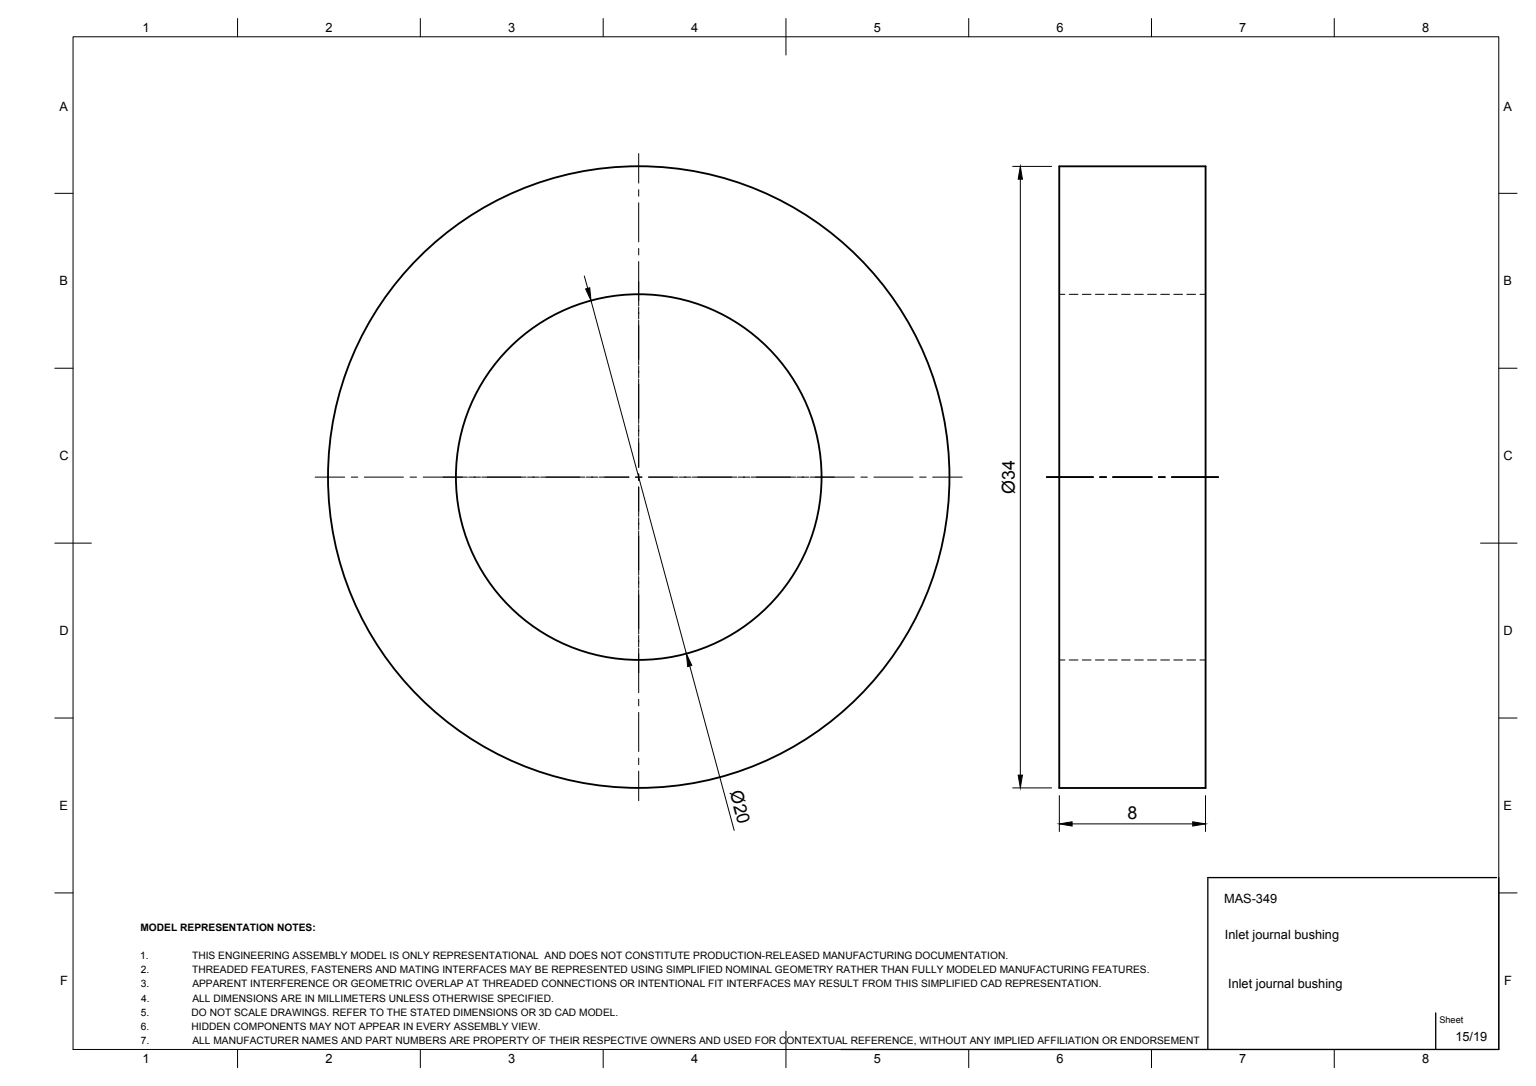
ISO-10303-21;
HEADER;
/* Generated by software containing ST-Developer
 * from STEP Tools, Inc. (www.steptools.com) 
 */

FILE_DESCRIPTION(
/* description */ ('Independent two-stage semi-open centrifugal-pump CAD. Shared impeller
s, open-machinable return casings, removable diaphragms, bronze wear/j
ournal rings, volume-preserving seal instances, retained keyed shaft, 
opposed mechanical face rings and partly threaded tie hardware. Native
 shaft rotation. Geometric topology/clearance only; flow/head/efficien
cy, pressure, cavitation, balance, preload, face loading and secondary
 seal fits/bonds, material/thermal/tolerance selection and life unassi
gned. External drive, coupling, anchors and piping bolts omitted.'),
/* implementation_level */ '2;1');

FILE_NAME(
/* name */ 'Inlet journal bushing.step',
/* time_stamp */ '2026-11-08T18:06:32-08:00',
/* author */ (''),
/* organization */ (''),
/* preprocessor_version */ 'ST-DEVELOPER v20.2',
/* originating_system */ 'Autodesk Translation Framework v15.17.0.0',
/* authorisation */ '');

FILE_SCHEMA (('AUTOMOTIVE_DESIGN { 1 0 10303 214 3 1 1 }'));
ENDSEC;

DATA;
#10=MECHANICAL_DESIGN_GEOMETRIC_PRESENTATION_REPRESENTATION('',(#404),#16687);
#366=SHAPE_REPRESENTATION_RELATIONSHIP('SRR','None',#16775,#385);
#385=ADVANCED_BREP_SHAPE_REPRESENTATION('',(#423),#16679);
#404=STYLED_ITEM('',(#16875),#423);
#423=MANIFOLD_SOLID_BREP('Body1',#6123);
#541=FACE_BOUND('',#1430,.T.);
#542=FACE_BOUND('',#1432,.T.);
#657=PLANE('',#6858);
#658=PLANE('',#6859);
#970=FACE_OUTER_BOUND('',#1427,.T.);
#971=FACE_OUTER_BOUND('',#1428,.T.);
#972=FACE_OUTER_BOUND('',#1429,.T.);
#973=FACE_OUTER_BOUND('',#1431,.T.);
#1427=EDGE_LOOP('',(#5293,#5294,#5295,#5296));
#1428=EDGE_LOOP('',(#5297,#5298,#5299,#5300));
#1429=EDGE_LOOP('',(#5301));
#1430=EDGE_LOOP('',(#5302));
#1431=EDGE_LOOP('',(#5303));
#1432=EDGE_LOOP('',(#5304));
#1810=LINE('',#15150,#2179);
#1811=LINE('',#15156,#2180);
#2179=VECTOR('',#8322,1.);
#2180=VECTOR('',#8329,1.7);
#2462=CIRCLE('',#6853,1.);
#2463=CIRCLE('',#6854,1.);
#2464=CIRCLE('',#6856,1.7);
#2465=CIRCLE('',#6857,1.7);
#2965=VERTEX_POINT('',#15147);
#2966=VERTEX_POINT('',#15149);
#2967=VERTEX_POINT('',#15153);
#2968=VERTEX_POINT('',#15155);
#3756=EDGE_CURVE('',#2965,#2965,#2462,.T.);
#3757=EDGE_CURVE('',#2965,#2966,#1810,.T.);
#3758=EDGE_CURVE('',#2966,#2966,#2463,.T.);
#3759=EDGE_CURVE('',#2967,#2967,#2464,.T.);
#3760=EDGE_CURVE('',#2967,#2968,#1811,.T.);
#3761=EDGE_CURVE('',#2968,#2968,#2465,.T.);
#5293=ORIENTED_EDGE('',*,*,#3756,.F.);
#5294=ORIENTED_EDGE('',*,*,#3757,.T.);
#5295=ORIENTED_EDGE('',*,*,#3758,.T.);
#5296=ORIENTED_EDGE('',*,*,#3757,.F.);
#5297=ORIENTED_EDGE('',*,*,#3759,.F.);
#5298=ORIENTED_EDGE('',*,*,#3760,.T.);
#5299=ORIENTED_EDGE('',*,*,#3761,.T.);
#5300=ORIENTED_EDGE('',*,*,#3760,.F.);
#5301=ORIENTED_EDGE('',*,*,#3759,.T.);
#5302=ORIENTED_EDGE('',*,*,#3756,.T.);
#5303=ORIENTED_EDGE('',*,*,#3761,.F.);
#5304=ORIENTED_EDGE('',*,*,#3758,.F.);
#5734=CYLINDRICAL_SURFACE('',#6852,1.);
#5735=CYLINDRICAL_SURFACE('',#6855,1.7);
#6049=ADVANCED_FACE('',(#970),#5734,.F.);
#6050=ADVANCED_FACE('',(#971),#5735,.T.);
#6051=ADVANCED_FACE('',(#972,#541),#657,.T.);
#6052=ADVANCED_FACE('',(#973,#542),#658,.F.);
#6123=CLOSED_SHELL('',(#6049,#6050,#6051,#6052));
#6851=AXIS2_PLACEMENT_3D('',#15145,#8316,#8317);
#6852=AXIS2_PLACEMENT_3D('',#15146,#8318,#8319);
#6853=AXIS2_PLACEMENT_3D('',#15148,#8320,#8321);
#6854=AXIS2_PLACEMENT_3D('',#15151,#8323,#8324);
#6855=AXIS2_PLACEMENT_3D('',#15152,#8325,#8326);
#6856=AXIS2_PLACEMENT_3D('',#15154,#8327,#8328);
#6857=AXIS2_PLACEMENT_3D('',#15157,#8330,#8331);
#6858=AXIS2_PLACEMENT_3D('',#15158,#8332,#8333);
#6859=AXIS2_PLACEMENT_3D('',#15159,#8334,#8335);
#8316=DIRECTION('axis',(0.,0.,1.));
#8317=DIRECTION('refdir',(1.,0.,0.));
#8318=DIRECTION('center_axis',(0.,0.,1.));
#8319=DIRECTION('ref_axis',(1.,0.,0.));
#8320=DIRECTION('center_axis',(0.,0.,-1.));
#8321=DIRECTION('ref_axis',(1.,0.,0.));
#8322=DIRECTION('',(0.,0.,-1.));
#8323=DIRECTION('center_axis',(0.,0.,-1.));
#8324=DIRECTION('ref_axis',(1.,0.,0.));
#8325=DIRECTION('center_axis',(0.,0.,1.));
#8326=DIRECTION('ref_axis',(1.,0.,0.));
#8327=DIRECTION('center_axis',(0.,0.,1.));
#8328=DIRECTION('ref_axis',(1.,0.,0.));
#8329=DIRECTION('',(0.,0.,-1.));
#8330=DIRECTION('center_axis',(0.,0.,1.));
#8331=DIRECTION('ref_axis',(1.,0.,0.));
#8332=DIRECTION('center_axis',(0.,0.,1.));
#8333=DIRECTION('ref_axis',(1.,0.,0.));
#8334=DIRECTION('center_axis',(0.,0.,1.));
#8335=DIRECTION('ref_axis',(1.,0.,0.));
#15145=CARTESIAN_POINT('',(0.,0.,0.));
#15146=CARTESIAN_POINT('Origin',(0.,0.,0.));
#15147=CARTESIAN_POINT('',(-1.,-1.22464679914735E-16,0.8));
#15148=CARTESIAN_POINT('Origin',(0.,0.,0.8));
#15149=CARTESIAN_POINT('',(-1.,-1.22464679914735E-16,0.));
#15150=CARTESIAN_POINT('',(-1.,-1.22464679914735E-16,0.));
#15151=CARTESIAN_POINT('Origin',(0.,0.,0.));
#15152=CARTESIAN_POINT('Origin',(0.,0.,0.));
#15153=CARTESIAN_POINT('',(-1.7,-2.0818995585505E-16,0.8));
#15154=CARTESIAN_POINT('Origin',(0.,0.,0.8));
#15155=CARTESIAN_POINT('',(-1.7,-2.0818995585505E-16,0.));
#15156=CARTESIAN_POINT('',(-1.7,-2.0818995585505E-16,0.));
#15157=CARTESIAN_POINT('Origin',(0.,0.,0.));
#15158=CARTESIAN_POINT('Origin',(0.,0.,0.8));
#15159=CARTESIAN_POINT('Origin',(0.,0.,0.));
#16658=UNCERTAINTY_MEASURE_WITH_UNIT(LENGTH_MEASURE(0.001),#16688,
'DISTANCE_ACCURACY_VALUE',
'Maximum model space distance between geometric entities at asserted c
onnectivities');
#16666=UNCERTAINTY_MEASURE_WITH_UNIT(LENGTH_MEASURE(0.001),#16688,
'DISTANCE_ACCURACY_VALUE',
'Maximum model space distance between geometric entities at asserted c
onnectivities');
#16679=(
GEOMETRIC_REPRESENTATION_CONTEXT(3)
GLOBAL_UNCERTAINTY_ASSIGNED_CONTEXT((#16658))
GLOBAL_UNIT_ASSIGNED_CONTEXT((#16688,#16690,#16691))
REPRESENTATION_CONTEXT('','3D')
);
#16687=(
GEOMETRIC_REPRESENTATION_CONTEXT(3)
GLOBAL_UNCERTAINTY_ASSIGNED_CONTEXT((#16666))
GLOBAL_UNIT_ASSIGNED_CONTEXT((#16688,#16690,#16691))
REPRESENTATION_CONTEXT('','3D')
);
#16688=(
LENGTH_UNIT()
NAMED_UNIT(*)
SI_UNIT(.CENTI.,.METRE.)
);
#16690=(
NAMED_UNIT(*)
PLANE_ANGLE_UNIT()
SI_UNIT($,.RADIAN.)
);
#16691=(
NAMED_UNIT(*)
SI_UNIT($,.STERADIAN.)
SOLID_ANGLE_UNIT()
);
#16704=SHAPE_DEFINITION_REPRESENTATION(#16724,#16775);
#16724=PRODUCT_DEFINITION_SHAPE('',$,#16796);
#16775=SHAPE_REPRESENTATION('',(#6851),#16679);
#16783=PRODUCT_DEFINITION_CONTEXT('part definition',#16845,'design');
#16796=PRODUCT_DEFINITION('Inlet journal bushing',
'Inlet journal bushing',#16816,#16783);
#16816=PRODUCT_DEFINITION_FORMATION('',$,#16859);
#16845=APPLICATION_CONTEXT(
'Core Data for Automotive Mechanical Design Process');
#16846=PRODUCT_CONTEXT('part definition',#16845,'mechanical');
#16859=PRODUCT('Inlet journal bushing','Inlet journal bushing',$,(#16846));
#16875=PRESENTATION_STYLE_ASSIGNMENT((#16890));
#16890=SURFACE_STYLE_USAGE(.BOTH.,#16905);
#16905=SURFACE_SIDE_STYLE('',(#16920));
#16920=SURFACE_STYLE_FILL_AREA(#16935);
#16935=FILL_AREA_STYLE('Journal gray',(#16950));
#16950=FILL_AREA_STYLE_COLOUR('Journal gray',#16965);
#16965=COLOUR_RGB('Journal gray',0.725490196078431,0.752941176470588,0.792156862745098);
ENDSEC;
END-ISO-10303-21;
